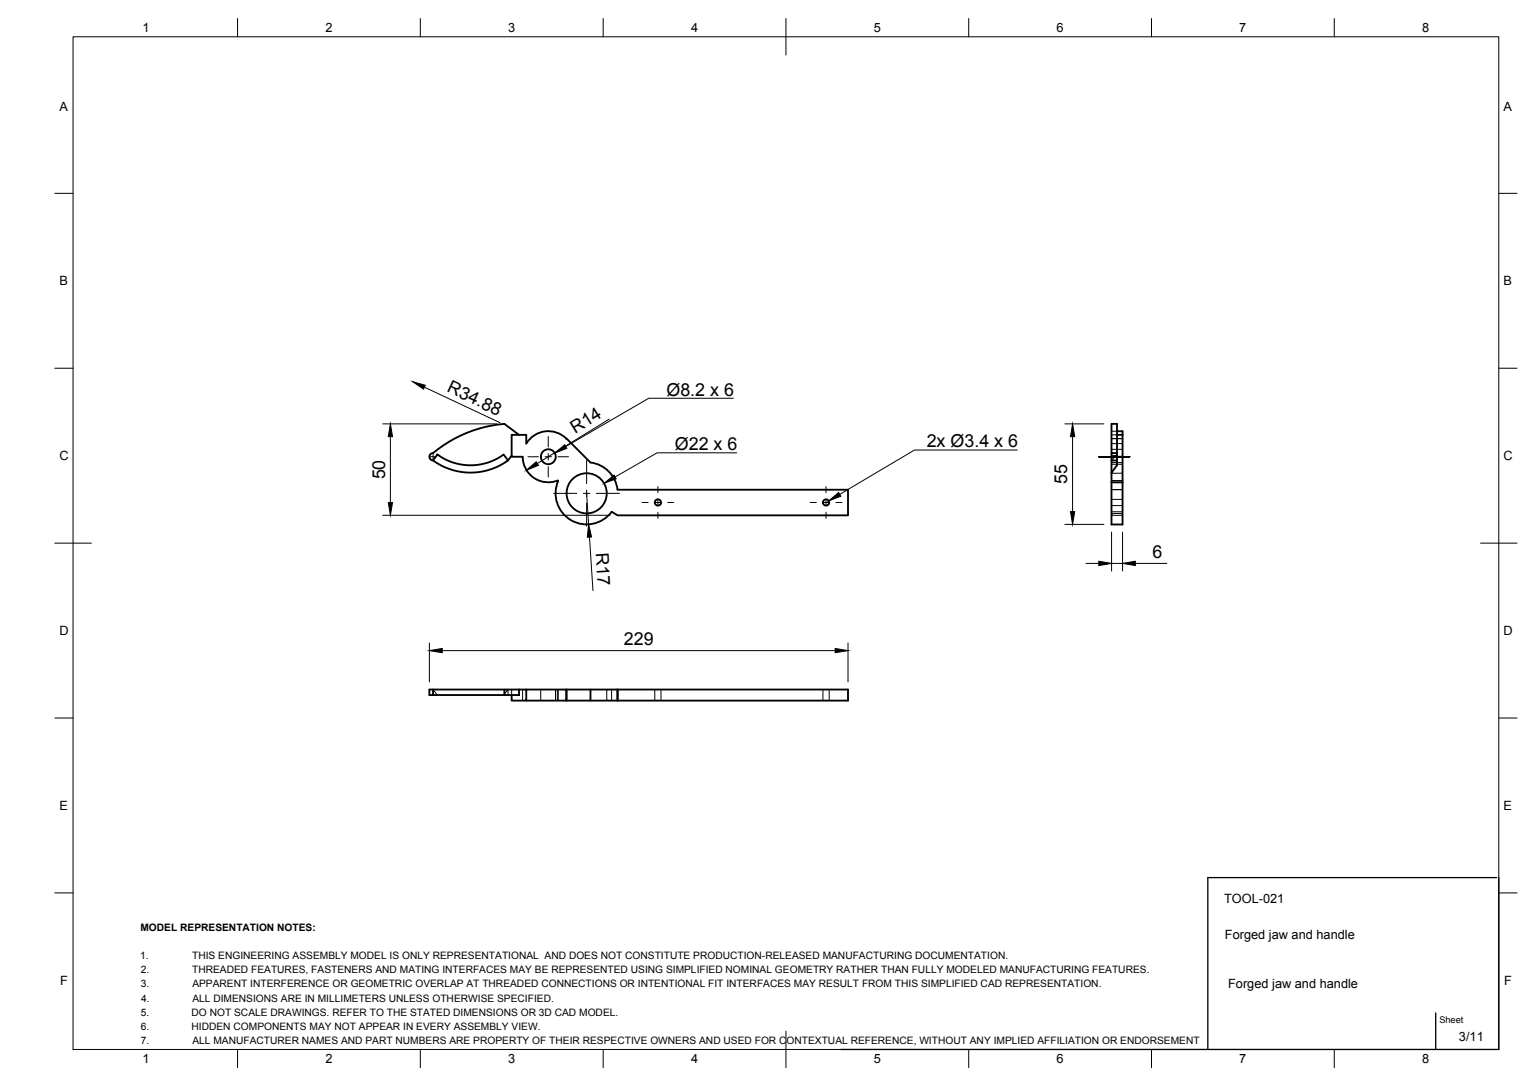
ISO-10303-21;
HEADER;
/* Generated by software containing ST-Developer
 * from STEP Tools, Inc. (www.steptools.com) 
 */

FILE_DESCRIPTION(
/* description */ (''),
/* implementation_level */ '2;1');

FILE_NAME(
/* name */ 'Forged jaw and handle.step',
/* time_stamp */ '2026-11-10T09:05:57-08:00',
/* author */ (''),
/* organization */ (''),
/* preprocessor_version */ 'ST-DEVELOPER v20.2',
/* originating_system */ 'Autodesk Translation Framework v15.17.0.0',
/* authorisation */ '');

FILE_SCHEMA (('AUTOMOTIVE_DESIGN { 1 0 10303 214 3 1 1 }'));
ENDSEC;

DATA;
#10=MECHANICAL_DESIGN_GEOMETRIC_PRESENTATION_REPRESENTATION('',(#565),#19618);
#545=SHAPE_REPRESENTATION_RELATIONSHIP('SRR','None',#19664,#555);
#555=ADVANCED_BREP_SHAPE_REPRESENTATION('',(#575),#19607);
#565=STYLED_ITEM('',(#19728),#575);
#575=MANIFOLD_SOLID_BREP('Body1',#7103);
#585=TOROIDAL_SURFACE('',#7263,1.2,0.1);
#586=TOROIDAL_SURFACE('',#7273,1.2,0.1);
#589=FACE_BOUND('',#1242,.T.);
#590=FACE_BOUND('',#1243,.T.);
#591=FACE_BOUND('',#1244,.T.);
#592=FACE_BOUND('',#1245,.T.);
#593=FACE_BOUND('',#1249,.T.);
#594=FACE_BOUND('',#1250,.T.);
#595=FACE_BOUND('',#1251,.T.);
#596=FACE_BOUND('',#1252,.T.);
#660=CONICAL_SURFACE('',#7236,3.28832599394285,0.927295218001612);
#662=PLANE('',#7235);
#663=PLANE('',#7239);
#664=PLANE('',#7240);
#665=PLANE('',#7241);
#666=PLANE('',#7248);
#667=PLANE('',#7249);
#668=PLANE('',#7250);
#669=PLANE('',#7251);
#670=PLANE('',#7252);
#671=PLANE('',#7259);
#672=PLANE('',#7270);
#673=PLANE('',#7277);
#674=PLANE('',#7278);
#675=PLANE('',#7279);
#676=PLANE('',#7280);
#677=PLANE('',#7281);
#678=PLANE('',#7282);
#679=PLANE('',#7283);
#680=PLANE('',#7284);
#821=FACE_OUTER_BOUND('',#1224,.T.);
#822=FACE_OUTER_BOUND('',#1225,.T.);
#823=FACE_OUTER_BOUND('',#1226,.T.);
#824=FACE_OUTER_BOUND('',#1227,.T.);
#825=FACE_OUTER_BOUND('',#1228,.T.);
#826=FACE_OUTER_BOUND('',#1229,.T.);
#827=FACE_OUTER_BOUND('',#1230,.T.);
#828=FACE_OUTER_BOUND('',#1231,.T.);
#829=FACE_OUTER_BOUND('',#1232,.T.);
#830=FACE_OUTER_BOUND('',#1233,.T.);
#831=FACE_OUTER_BOUND('',#1234,.T.);
#832=FACE_OUTER_BOUND('',#1235,.T.);
#833=FACE_OUTER_BOUND('',#1236,.T.);
#834=FACE_OUTER_BOUND('',#1237,.T.);
#835=FACE_OUTER_BOUND('',#1238,.T.);
#836=FACE_OUTER_BOUND('',#1239,.T.);
#837=FACE_OUTER_BOUND('',#1240,.T.);
#838=FACE_OUTER_BOUND('',#1241,.T.);
#839=FACE_OUTER_BOUND('',#1246,.T.);
#840=FACE_OUTER_BOUND('',#1247,.T.);
#841=FACE_OUTER_BOUND('',#1248,.T.);
#842=FACE_OUTER_BOUND('',#1253,.T.);
#843=FACE_OUTER_BOUND('',#1254,.T.);
#844=FACE_OUTER_BOUND('',#1255,.T.);
#845=FACE_OUTER_BOUND('',#1256,.T.);
#846=FACE_OUTER_BOUND('',#1257,.T.);
#847=FACE_OUTER_BOUND('',#1258,.T.);
#848=FACE_OUTER_BOUND('',#1259,.T.);
#849=FACE_OUTER_BOUND('',#1260,.T.);
#850=FACE_OUTER_BOUND('',#1261,.T.);
#851=FACE_OUTER_BOUND('',#1262,.T.);
#852=FACE_OUTER_BOUND('',#1263,.T.);
#1224=EDGE_LOOP('',(#4504,#4505,#4506,#4507));
#1225=EDGE_LOOP('',(#4508,#4509,#4510,#4511));
#1226=EDGE_LOOP('',(#4512,#4513,#4514,#4515));
#1227=EDGE_LOOP('',(#4516,#4517,#4518));
#1228=EDGE_LOOP('',(#4519,#4520,#4521,#4522));
#1229=EDGE_LOOP('',(#4523,#4524,#4525));
#1230=EDGE_LOOP('',(#4526,#4527,#4528,#4529));
#1231=EDGE_LOOP('',(#4530,#4531,#4532,#4533));
#1232=EDGE_LOOP('',(#4534,#4535,#4536,#4537));
#1233=EDGE_LOOP('',(#4538,#4539,#4540,#4541));
#1234=EDGE_LOOP('',(#4542,#4543,#4544,#4545,#4546,#4547,#4548,#4549,#4550));
#1235=EDGE_LOOP('',(#4551,#4552,#4553,#4554,#4555,#4556));
#1236=EDGE_LOOP('',(#4557,#4558,#4559,#4560,#4561,#4562));
#1237=EDGE_LOOP('',(#4563,#4564,#4565,#4566));
#1238=EDGE_LOOP('',(#4567,#4568,#4569,#4570));
#1239=EDGE_LOOP('',(#4571,#4572,#4573,#4574));
#1240=EDGE_LOOP('',(#4575,#4576,#4577,#4578));
#1241=EDGE_LOOP('',(#4579,#4580,#4581,#4582,#4583,#4584,#4585,#4586,#4587,
#4588,#4589,#4590,#4591,#4592,#4593,#4594));
#1242=EDGE_LOOP('',(#4595));
#1243=EDGE_LOOP('',(#4596));
#1244=EDGE_LOOP('',(#4597));
#1245=EDGE_LOOP('',(#4598));
#1246=EDGE_LOOP('',(#4599,#4600,#4601,#4602));
#1247=EDGE_LOOP('',(#4603,#4604,#4605,#4606,#4607));
#1248=EDGE_LOOP('',(#4608,#4609,#4610,#4611,#4612,#4613,#4614,#4615,#4616,
#4617,#4618,#4619,#4620,#4621,#4622,#4623,#4624,#4625,#4626,#4627,#4628));
#1249=EDGE_LOOP('',(#4629));
#1250=EDGE_LOOP('',(#4630));
#1251=EDGE_LOOP('',(#4631));
#1252=EDGE_LOOP('',(#4632));
#1253=EDGE_LOOP('',(#4633,#4634,#4635,#4636,#4637));
#1254=EDGE_LOOP('',(#4638,#4639,#4640,#4641));
#1255=EDGE_LOOP('',(#4642,#4643,#4644,#4645));
#1256=EDGE_LOOP('',(#4646,#4647,#4648,#4649));
#1257=EDGE_LOOP('',(#4650,#4651,#4652,#4653));
#1258=EDGE_LOOP('',(#4654,#4655,#4656,#4657));
#1259=EDGE_LOOP('',(#4658,#4659,#4660,#4661));
#1260=EDGE_LOOP('',(#4662,#4663,#4664,#4665));
#1261=EDGE_LOOP('',(#4666,#4667,#4668,#4669));
#1262=EDGE_LOOP('',(#4670,#4671,#4672,#4673));
#1263=EDGE_LOOP('',(#4674,#4675,#4676,#4677));
#1698=LINE('',#9324,#2157);
#1699=LINE('',#9330,#2158);
#1700=LINE('',#9336,#2159);
#1701=LINE('',#9341,#2160);
#1702=LINE('',#9343,#2161);
#1703=LINE('',#9344,#2162);
#1704=LINE('',#9348,#2163);
#1705=LINE('',#9353,#2164);
#1706=LINE('',#9354,#2165);
#1707=LINE('',#9358,#2166);
#1708=LINE('',#9359,#2167);
#1709=LINE('',#9360,#2168);
#1710=LINE('',#9364,#2169);
#1711=LINE('',#9366,#2170);
#1712=LINE('',#9368,#2171);
#1713=LINE('',#9369,#2172);
#1714=LINE('',#9375,#2173);
#1715=LINE('',#9381,#2174);
#1716=LINE('',#9382,#2175);
#1717=LINE('',#9385,#2176);
#1718=LINE('',#9387,#2177);
#1719=LINE('',#9389,#2178);
#1720=LINE('',#9390,#2179);
#1721=LINE('',#9393,#2180);
#1722=LINE('',#9395,#2181);
#1723=LINE('',#9396,#2182);
#1724=LINE('',#9400,#2183);
#1725=LINE('',#9401,#2184);
#1726=LINE('',#9402,#2185);
#1727=LINE('',#9406,#2186);
#1728=LINE('',#9407,#2187);
#1729=LINE('',#9408,#2188);
#1730=LINE('',#9413,#2189);
#1731=LINE('',#9419,#2190);
#1732=LINE('',#9423,#2191);
#1733=LINE('',#9427,#2192);
#1734=LINE('',#9429,#2193);
#1735=LINE('',#9431,#2194);
#1736=LINE('',#9433,#2195);
#1737=LINE('',#9435,#2196);
#1738=LINE('',#9439,#2197);
#1739=LINE('',#9440,#2198);
#1740=LINE('',#9454,#2199);
#1741=LINE('',#9457,#2200);
#1742=LINE('',#9459,#2201);
#1743=LINE('',#9463,#2202);
#1744=LINE('',#9465,#2203);
#1745=LINE('',#9467,#2204);
#1746=LINE('',#9469,#2205);
#1747=LINE('',#9471,#2206);
#1748=LINE('',#9474,#2207);
#1749=LINE('',#9478,#2208);
#1750=LINE('',#9479,#2209);
#1751=LINE('',#9481,#2210);
#1752=LINE('',#9482,#2211);
#1753=LINE('',#9484,#2212);
#1754=LINE('',#9486,#2213);
#1755=LINE('',#9489,#2214);
#1756=LINE('',#9492,#2215);
#1757=LINE('',#9494,#2216);
#2157=VECTOR('',#7777,0.17);
#2158=VECTOR('',#7784,0.17);
#2159=VECTOR('',#7791,0.41);
#2160=VECTOR('',#7796,1.);
#2161=VECTOR('',#7797,1.);
#2162=VECTOR('',#7798,1.);
#2163=VECTOR('',#7801,1.);
#2164=VECTOR('',#7808,1.);
#2165=VECTOR('',#7809,1.);
#2166=VECTOR('',#7812,1.);
#2167=VECTOR('',#7813,1.);
#2168=VECTOR('',#7814,1.);
#2169=VECTOR('',#7817,1.);
#2170=VECTOR('',#7818,1.);
#2171=VECTOR('',#7819,1.);
#2172=VECTOR('',#7820,1.);
#2173=VECTOR('',#7827,1.);
#2174=VECTOR('',#7836,1.);
#2175=VECTOR('',#7837,1.);
#2176=VECTOR('',#7840,1.);
#2177=VECTOR('',#7841,1.);
#2178=VECTOR('',#7842,1.);
#2179=VECTOR('',#7843,1.);
#2180=VECTOR('',#7846,1.);
#2181=VECTOR('',#7847,1.);
#2182=VECTOR('',#7848,1.);
#2183=VECTOR('',#7851,1.);
#2184=VECTOR('',#7852,1.);
#2185=VECTOR('',#7853,1.);
#2186=VECTOR('',#7856,1.);
#2187=VECTOR('',#7857,1.);
#2188=VECTOR('',#7858,1.);
#2189=VECTOR('',#7863,1.);
#2190=VECTOR('',#7870,1.);
#2191=VECTOR('',#7875,1.);
#2192=VECTOR('',#7878,1.);
#2193=VECTOR('',#7879,1.);
#2194=VECTOR('',#7880,1.);
#2195=VECTOR('',#7881,1.);
#2196=VECTOR('',#7882,1.);
#2197=VECTOR('',#7885,1.);
#2198=VECTOR('',#7886,1.);
#2199=VECTOR('',#7903,1.1);
#2200=VECTOR('',#7906,1.);
#2201=VECTOR('',#7907,1.);
#2202=VECTOR('',#7910,1.);
#2203=VECTOR('',#7911,1.);
#2204=VECTOR('',#7912,1.);
#2205=VECTOR('',#7913,1.);
#2206=VECTOR('',#7914,1.);
#2207=VECTOR('',#7917,1.);
#2208=VECTOR('',#7924,1.);
#2209=VECTOR('',#7925,1.);
#2210=VECTOR('',#7928,1.);
#2211=VECTOR('',#7929,1.);
#2212=VECTOR('',#7932,1.);
#2213=VECTOR('',#7935,1.);
#2214=VECTOR('',#7940,1.);
#2215=VECTOR('',#7945,1.);
#2216=VECTOR('',#7948,1.);
#2616=CIRCLE('',#7227,0.17);
#2617=CIRCLE('',#7228,0.17);
#2618=CIRCLE('',#7230,0.17);
#2619=CIRCLE('',#7231,0.17);
#2620=CIRCLE('',#7233,0.41);
#2621=CIRCLE('',#7234,0.41);
#2622=CIRCLE('',#7237,3.48832599394285);
#2623=CIRCLE('',#7238,3.08832599394285);
#2624=CIRCLE('',#7243,0.2);
#2625=CIRCLE('',#7244,0.2);
#2626=CIRCLE('',#7246,6.99668559332711);
#2627=CIRCLE('',#7247,6.99668559332711);
#2628=CIRCLE('',#7254,1.4);
#2629=CIRCLE('',#7255,1.4);
#2630=CIRCLE('',#7257,1.4);
#2631=CIRCLE('',#7258,1.4);
#2632=CIRCLE('',#7260,1.7);
#2633=CIRCLE('',#7261,1.7);
#2634=CIRCLE('',#7262,1.2);
#2635=CIRCLE('',#7264,1.2);
#2636=CIRCLE('',#7265,0.1);
#2637=CIRCLE('',#7266,1.1);
#2638=CIRCLE('',#7268,1.1);
#2639=CIRCLE('',#7269,1.1);
#2640=CIRCLE('',#7271,1.7);
#2641=CIRCLE('',#7272,1.7);
#2642=CIRCLE('',#7274,0.1);
#2810=VERTEX_POINT('',#9321);
#2811=VERTEX_POINT('',#9323);
#2812=VERTEX_POINT('',#9327);
#2813=VERTEX_POINT('',#9329);
#2814=VERTEX_POINT('',#9333);
#2815=VERTEX_POINT('',#9335);
#2816=VERTEX_POINT('',#9339);
#2817=VERTEX_POINT('',#9340);
#2818=VERTEX_POINT('',#9342);
#2819=VERTEX_POINT('',#9346);
#2820=VERTEX_POINT('',#9347);
#2821=VERTEX_POINT('',#9352);
#2822=VERTEX_POINT('',#9356);
#2823=VERTEX_POINT('',#9357);
#2824=VERTEX_POINT('',#9362);
#2825=VERTEX_POINT('',#9363);
#2826=VERTEX_POINT('',#9365);
#2827=VERTEX_POINT('',#9367);
#2828=VERTEX_POINT('',#9371);
#2829=VERTEX_POINT('',#9373);
#2830=VERTEX_POINT('',#9380);
#2831=VERTEX_POINT('',#9384);
#2832=VERTEX_POINT('',#9386);
#2833=VERTEX_POINT('',#9388);
#2834=VERTEX_POINT('',#9392);
#2835=VERTEX_POINT('',#9394);
#2836=VERTEX_POINT('',#9398);
#2837=VERTEX_POINT('',#9399);
#2838=VERTEX_POINT('',#9404);
#2839=VERTEX_POINT('',#9405);
#2840=VERTEX_POINT('',#9410);
#2841=VERTEX_POINT('',#9412);
#2842=VERTEX_POINT('',#9416);
#2843=VERTEX_POINT('',#9418);
#2844=VERTEX_POINT('',#9422);
#2845=VERTEX_POINT('',#9424);
#2846=VERTEX_POINT('',#9426);
#2847=VERTEX_POINT('',#9428);
#2848=VERTEX_POINT('',#9430);
#2849=VERTEX_POINT('',#9432);
#2850=VERTEX_POINT('',#9434);
#2851=VERTEX_POINT('',#9436);
#2852=VERTEX_POINT('',#9438);
#2853=VERTEX_POINT('',#9441);
#2854=VERTEX_POINT('',#9444);
#2855=VERTEX_POINT('',#9446);
#2856=VERTEX_POINT('',#9450);
#2857=VERTEX_POINT('',#9451);
#2858=VERTEX_POINT('',#9456);
#2859=VERTEX_POINT('',#9458);
#2860=VERTEX_POINT('',#9460);
#2861=VERTEX_POINT('',#9462);
#2862=VERTEX_POINT('',#9464);
#2863=VERTEX_POINT('',#9466);
#2864=VERTEX_POINT('',#9468);
#2865=VERTEX_POINT('',#9470);
#2866=VERTEX_POINT('',#9472);
#3477=EDGE_CURVE('',#2810,#2810,#2616,.T.);
#3478=EDGE_CURVE('',#2810,#2811,#1698,.T.);
#3479=EDGE_CURVE('',#2811,#2811,#2617,.T.);
#3480=EDGE_CURVE('',#2812,#2812,#2618,.T.);
#3481=EDGE_CURVE('',#2812,#2813,#1699,.T.);
#3482=EDGE_CURVE('',#2813,#2813,#2619,.T.);
#3483=EDGE_CURVE('',#2814,#2814,#2620,.T.);
#3484=EDGE_CURVE('',#2814,#2815,#1700,.T.);
#3485=EDGE_CURVE('',#2815,#2815,#2621,.T.);
#3486=EDGE_CURVE('',#2816,#2817,#1701,.T.);
#3487=EDGE_CURVE('',#2818,#2816,#1702,.T.);
#3488=EDGE_CURVE('',#2818,#2817,#1703,.T.);
#3489=EDGE_CURVE('',#2819,#2820,#1704,.T.);
#3490=EDGE_CURVE('',#2819,#2818,#2622,.T.);
#3491=EDGE_CURVE('',#2820,#2816,#2623,.T.);
#3492=EDGE_CURVE('',#2821,#2820,#1705,.T.);
#3493=EDGE_CURVE('',#2819,#2821,#1706,.T.);
#3494=EDGE_CURVE('',#2822,#2823,#1707,.T.);
#3495=EDGE_CURVE('',#2817,#2822,#1708,.T.);
#3496=EDGE_CURVE('',#2823,#2818,#1709,.T.);
#3497=EDGE_CURVE('',#2824,#2825,#1710,.T.);
#3498=EDGE_CURVE('',#2824,#2826,#1711,.T.);
#3499=EDGE_CURVE('',#2827,#2826,#1712,.T.);
#3500=EDGE_CURVE('',#2825,#2827,#1713,.T.);
#3501=EDGE_CURVE('',#2828,#2819,#2624,.T.);
#3502=EDGE_CURVE('',#2829,#2821,#2625,.T.);
#3503=EDGE_CURVE('',#2828,#2829,#1714,.T.);
#3504=EDGE_CURVE('',#2824,#2828,#2626,.T.);
#3505=EDGE_CURVE('',#2826,#2829,#2627,.T.);
#3506=EDGE_CURVE('',#2830,#2822,#1715,.T.);
#3507=EDGE_CURVE('',#2827,#2830,#1716,.T.);
#3508=EDGE_CURVE('',#2830,#2831,#1717,.T.);
#3509=EDGE_CURVE('',#2832,#2831,#1718,.T.);
#3510=EDGE_CURVE('',#2833,#2832,#1719,.T.);
#3511=EDGE_CURVE('',#2825,#2833,#1720,.T.);
#3512=EDGE_CURVE('',#2834,#2823,#1721,.T.);
#3513=EDGE_CURVE('',#2834,#2835,#1722,.T.);
#3514=EDGE_CURVE('',#2831,#2835,#1723,.T.);
#3515=EDGE_CURVE('',#2836,#2837,#1724,.T.);
#3516=EDGE_CURVE('',#2835,#2836,#1725,.T.);
#3517=EDGE_CURVE('',#2837,#2834,#1726,.T.);
#3518=EDGE_CURVE('',#2838,#2839,#1727,.T.);
#3519=EDGE_CURVE('',#2833,#2838,#1728,.T.);
#3520=EDGE_CURVE('',#2839,#2832,#1729,.T.);
#3521=EDGE_CURVE('',#2837,#2840,#2628,.T.);
#3522=EDGE_CURVE('',#2840,#2841,#1730,.T.);
#3523=EDGE_CURVE('',#2836,#2841,#2629,.T.);
#3524=EDGE_CURVE('',#2842,#2839,#2630,.T.);
#3525=EDGE_CURVE('',#2842,#2843,#1731,.T.);
#3526=EDGE_CURVE('',#2843,#2838,#2631,.T.);
#3527=EDGE_CURVE('',#2841,#2844,#1732,.T.);
#3528=EDGE_CURVE('',#2844,#2845,#2632,.T.);
#3529=EDGE_CURVE('',#2845,#2846,#1733,.T.);
#3530=EDGE_CURVE('',#2846,#2847,#1734,.T.);
#3531=EDGE_CURVE('',#2847,#2848,#1735,.T.);
#3532=EDGE_CURVE('',#2848,#2849,#1736,.T.);
#3533=EDGE_CURVE('',#2849,#2850,#1737,.T.);
#3534=EDGE_CURVE('',#2850,#2851,#2633,.T.);
#3535=EDGE_CURVE('',#2851,#2852,#1738,.T.);
#3536=EDGE_CURVE('',#2852,#2842,#1739,.T.);
#3537=EDGE_CURVE('',#2853,#2853,#2634,.T.);
#3538=EDGE_CURVE('',#2854,#2854,#2635,.T.);
#3539=EDGE_CURVE('',#2854,#2855,#2636,.T.);
#3540=EDGE_CURVE('',#2855,#2855,#2637,.T.);
#3541=EDGE_CURVE('',#2856,#2857,#2638,.T.);
#3542=EDGE_CURVE('',#2857,#2856,#2639,.T.);
#3543=EDGE_CURVE('',#2857,#2855,#1740,.T.);
#3544=EDGE_CURVE('',#2858,#2843,#1741,.T.);
#3545=EDGE_CURVE('',#2859,#2858,#1742,.T.);
#3546=EDGE_CURVE('',#2860,#2859,#2640,.T.);
#3547=EDGE_CURVE('',#2861,#2860,#1743,.T.);
#3548=EDGE_CURVE('',#2862,#2861,#1744,.T.);
#3549=EDGE_CURVE('',#2863,#2862,#1745,.T.);
#3550=EDGE_CURVE('',#2864,#2863,#1746,.T.);
#3551=EDGE_CURVE('',#2865,#2864,#1747,.T.);
#3552=EDGE_CURVE('',#2866,#2865,#2641,.T.);
#3553=EDGE_CURVE('',#2840,#2866,#1748,.T.);
#3554=EDGE_CURVE('',#2853,#2856,#2642,.T.);
#3555=EDGE_CURVE('',#2851,#2859,#1749,.T.);
#3556=EDGE_CURVE('',#2860,#2850,#1750,.T.);
#3557=EDGE_CURVE('',#2866,#2844,#1751,.T.);
#3558=EDGE_CURVE('',#2845,#2865,#1752,.T.);
#3559=EDGE_CURVE('',#2864,#2846,#1753,.T.);
#3560=EDGE_CURVE('',#2861,#2849,#1754,.T.);
#3561=EDGE_CURVE('',#2858,#2852,#1755,.T.);
#3562=EDGE_CURVE('',#2862,#2848,#1756,.T.);
#3563=EDGE_CURVE('',#2863,#2847,#1757,.T.);
#4504=ORIENTED_EDGE('',*,*,#3477,.F.);
#4505=ORIENTED_EDGE('',*,*,#3478,.T.);
#4506=ORIENTED_EDGE('',*,*,#3479,.F.);
#4507=ORIENTED_EDGE('',*,*,#3478,.F.);
#4508=ORIENTED_EDGE('',*,*,#3480,.F.);
#4509=ORIENTED_EDGE('',*,*,#3481,.T.);
#4510=ORIENTED_EDGE('',*,*,#3482,.F.);
#4511=ORIENTED_EDGE('',*,*,#3481,.F.);
#4512=ORIENTED_EDGE('',*,*,#3483,.F.);
#4513=ORIENTED_EDGE('',*,*,#3484,.T.);
#4514=ORIENTED_EDGE('',*,*,#3485,.F.);
#4515=ORIENTED_EDGE('',*,*,#3484,.F.);
#4516=ORIENTED_EDGE('',*,*,#3486,.F.);
#4517=ORIENTED_EDGE('',*,*,#3487,.F.);
#4518=ORIENTED_EDGE('',*,*,#3488,.T.);
#4519=ORIENTED_EDGE('',*,*,#3489,.F.);
#4520=ORIENTED_EDGE('',*,*,#3490,.T.);
#4521=ORIENTED_EDGE('',*,*,#3487,.T.);
#4522=ORIENTED_EDGE('',*,*,#3491,.F.);
#4523=ORIENTED_EDGE('',*,*,#3492,.F.);
#4524=ORIENTED_EDGE('',*,*,#3493,.F.);
#4525=ORIENTED_EDGE('',*,*,#3489,.T.);
#4526=ORIENTED_EDGE('',*,*,#3494,.F.);
#4527=ORIENTED_EDGE('',*,*,#3495,.F.);
#4528=ORIENTED_EDGE('',*,*,#3488,.F.);
#4529=ORIENTED_EDGE('',*,*,#3496,.F.);
#4530=ORIENTED_EDGE('',*,*,#3497,.F.);
#4531=ORIENTED_EDGE('',*,*,#3498,.T.);
#4532=ORIENTED_EDGE('',*,*,#3499,.F.);
#4533=ORIENTED_EDGE('',*,*,#3500,.F.);
#4534=ORIENTED_EDGE('',*,*,#3501,.T.);
#4535=ORIENTED_EDGE('',*,*,#3493,.T.);
#4536=ORIENTED_EDGE('',*,*,#3502,.F.);
#4537=ORIENTED_EDGE('',*,*,#3503,.F.);
#4538=ORIENTED_EDGE('',*,*,#3504,.T.);
#4539=ORIENTED_EDGE('',*,*,#3503,.T.);
#4540=ORIENTED_EDGE('',*,*,#3505,.F.);
#4541=ORIENTED_EDGE('',*,*,#3498,.F.);
#4542=ORIENTED_EDGE('',*,*,#3486,.T.);
#4543=ORIENTED_EDGE('',*,*,#3495,.T.);
#4544=ORIENTED_EDGE('',*,*,#3506,.F.);
#4545=ORIENTED_EDGE('',*,*,#3507,.F.);
#4546=ORIENTED_EDGE('',*,*,#3499,.T.);
#4547=ORIENTED_EDGE('',*,*,#3505,.T.);
#4548=ORIENTED_EDGE('',*,*,#3502,.T.);
#4549=ORIENTED_EDGE('',*,*,#3492,.T.);
#4550=ORIENTED_EDGE('',*,*,#3491,.T.);
#4551=ORIENTED_EDGE('',*,*,#3500,.T.);
#4552=ORIENTED_EDGE('',*,*,#3507,.T.);
#4553=ORIENTED_EDGE('',*,*,#3508,.T.);
#4554=ORIENTED_EDGE('',*,*,#3509,.F.);
#4555=ORIENTED_EDGE('',*,*,#3510,.F.);
#4556=ORIENTED_EDGE('',*,*,#3511,.F.);
#4557=ORIENTED_EDGE('',*,*,#3506,.T.);
#4558=ORIENTED_EDGE('',*,*,#3494,.T.);
#4559=ORIENTED_EDGE('',*,*,#3512,.F.);
#4560=ORIENTED_EDGE('',*,*,#3513,.T.);
#4561=ORIENTED_EDGE('',*,*,#3514,.F.);
#4562=ORIENTED_EDGE('',*,*,#3508,.F.);
#4563=ORIENTED_EDGE('',*,*,#3515,.F.);
#4564=ORIENTED_EDGE('',*,*,#3516,.F.);
#4565=ORIENTED_EDGE('',*,*,#3513,.F.);
#4566=ORIENTED_EDGE('',*,*,#3517,.F.);
#4567=ORIENTED_EDGE('',*,*,#3518,.F.);
#4568=ORIENTED_EDGE('',*,*,#3519,.F.);
#4569=ORIENTED_EDGE('',*,*,#3510,.T.);
#4570=ORIENTED_EDGE('',*,*,#3520,.F.);
#4571=ORIENTED_EDGE('',*,*,#3515,.T.);
#4572=ORIENTED_EDGE('',*,*,#3521,.T.);
#4573=ORIENTED_EDGE('',*,*,#3522,.T.);
#4574=ORIENTED_EDGE('',*,*,#3523,.F.);
#4575=ORIENTED_EDGE('',*,*,#3518,.T.);
#4576=ORIENTED_EDGE('',*,*,#3524,.F.);
#4577=ORIENTED_EDGE('',*,*,#3525,.T.);
#4578=ORIENTED_EDGE('',*,*,#3526,.T.);
#4579=ORIENTED_EDGE('',*,*,#3523,.T.);
#4580=ORIENTED_EDGE('',*,*,#3527,.T.);
#4581=ORIENTED_EDGE('',*,*,#3528,.T.);
#4582=ORIENTED_EDGE('',*,*,#3529,.T.);
#4583=ORIENTED_EDGE('',*,*,#3530,.T.);
#4584=ORIENTED_EDGE('',*,*,#3531,.T.);
#4585=ORIENTED_EDGE('',*,*,#3532,.T.);
#4586=ORIENTED_EDGE('',*,*,#3533,.T.);
#4587=ORIENTED_EDGE('',*,*,#3534,.T.);
#4588=ORIENTED_EDGE('',*,*,#3535,.T.);
#4589=ORIENTED_EDGE('',*,*,#3536,.T.);
#4590=ORIENTED_EDGE('',*,*,#3524,.T.);
#4591=ORIENTED_EDGE('',*,*,#3520,.T.);
#4592=ORIENTED_EDGE('',*,*,#3509,.T.);
#4593=ORIENTED_EDGE('',*,*,#3514,.T.);
#4594=ORIENTED_EDGE('',*,*,#3516,.T.);
#4595=ORIENTED_EDGE('',*,*,#3477,.T.);
#4596=ORIENTED_EDGE('',*,*,#3480,.T.);
#4597=ORIENTED_EDGE('',*,*,#3483,.T.);
#4598=ORIENTED_EDGE('',*,*,#3537,.F.);
#4599=ORIENTED_EDGE('',*,*,#3538,.T.);
#4600=ORIENTED_EDGE('',*,*,#3539,.T.);
#4601=ORIENTED_EDGE('',*,*,#3540,.T.);
#4602=ORIENTED_EDGE('',*,*,#3539,.F.);
#4603=ORIENTED_EDGE('',*,*,#3541,.F.);
#4604=ORIENTED_EDGE('',*,*,#3542,.F.);
#4605=ORIENTED_EDGE('',*,*,#3543,.T.);
#4606=ORIENTED_EDGE('',*,*,#3540,.F.);
#4607=ORIENTED_EDGE('',*,*,#3543,.F.);
#4608=ORIENTED_EDGE('',*,*,#3511,.T.);
#4609=ORIENTED_EDGE('',*,*,#3519,.T.);
#4610=ORIENTED_EDGE('',*,*,#3526,.F.);
#4611=ORIENTED_EDGE('',*,*,#3544,.F.);
#4612=ORIENTED_EDGE('',*,*,#3545,.F.);
#4613=ORIENTED_EDGE('',*,*,#3546,.F.);
#4614=ORIENTED_EDGE('',*,*,#3547,.F.);
#4615=ORIENTED_EDGE('',*,*,#3548,.F.);
#4616=ORIENTED_EDGE('',*,*,#3549,.F.);
#4617=ORIENTED_EDGE('',*,*,#3550,.F.);
#4618=ORIENTED_EDGE('',*,*,#3551,.F.);
#4619=ORIENTED_EDGE('',*,*,#3552,.F.);
#4620=ORIENTED_EDGE('',*,*,#3553,.F.);
#4621=ORIENTED_EDGE('',*,*,#3521,.F.);
#4622=ORIENTED_EDGE('',*,*,#3517,.T.);
#4623=ORIENTED_EDGE('',*,*,#3512,.T.);
#4624=ORIENTED_EDGE('',*,*,#3496,.T.);
#4625=ORIENTED_EDGE('',*,*,#3490,.F.);
#4626=ORIENTED_EDGE('',*,*,#3501,.F.);
#4627=ORIENTED_EDGE('',*,*,#3504,.F.);
#4628=ORIENTED_EDGE('',*,*,#3497,.T.);
#4629=ORIENTED_EDGE('',*,*,#3479,.T.);
#4630=ORIENTED_EDGE('',*,*,#3482,.T.);
#4631=ORIENTED_EDGE('',*,*,#3485,.T.);
#4632=ORIENTED_EDGE('',*,*,#3538,.F.);
#4633=ORIENTED_EDGE('',*,*,#3537,.T.);
#4634=ORIENTED_EDGE('',*,*,#3554,.T.);
#4635=ORIENTED_EDGE('',*,*,#3541,.T.);
#4636=ORIENTED_EDGE('',*,*,#3542,.T.);
#4637=ORIENTED_EDGE('',*,*,#3554,.F.);
#4638=ORIENTED_EDGE('',*,*,#3555,.F.);
#4639=ORIENTED_EDGE('',*,*,#3534,.F.);
#4640=ORIENTED_EDGE('',*,*,#3556,.F.);
#4641=ORIENTED_EDGE('',*,*,#3546,.T.);
#4642=ORIENTED_EDGE('',*,*,#3557,.F.);
#4643=ORIENTED_EDGE('',*,*,#3552,.T.);
#4644=ORIENTED_EDGE('',*,*,#3558,.F.);
#4645=ORIENTED_EDGE('',*,*,#3528,.F.);
#4646=ORIENTED_EDGE('',*,*,#3558,.T.);
#4647=ORIENTED_EDGE('',*,*,#3551,.T.);
#4648=ORIENTED_EDGE('',*,*,#3559,.T.);
#4649=ORIENTED_EDGE('',*,*,#3529,.F.);
#4650=ORIENTED_EDGE('',*,*,#3556,.T.);
#4651=ORIENTED_EDGE('',*,*,#3533,.F.);
#4652=ORIENTED_EDGE('',*,*,#3560,.F.);
#4653=ORIENTED_EDGE('',*,*,#3547,.T.);
#4654=ORIENTED_EDGE('',*,*,#3557,.T.);
#4655=ORIENTED_EDGE('',*,*,#3527,.F.);
#4656=ORIENTED_EDGE('',*,*,#3522,.F.);
#4657=ORIENTED_EDGE('',*,*,#3553,.T.);
#4658=ORIENTED_EDGE('',*,*,#3525,.F.);
#4659=ORIENTED_EDGE('',*,*,#3536,.F.);
#4660=ORIENTED_EDGE('',*,*,#3561,.F.);
#4661=ORIENTED_EDGE('',*,*,#3544,.T.);
#4662=ORIENTED_EDGE('',*,*,#3555,.T.);
#4663=ORIENTED_EDGE('',*,*,#3545,.T.);
#4664=ORIENTED_EDGE('',*,*,#3561,.T.);
#4665=ORIENTED_EDGE('',*,*,#3535,.F.);
#4666=ORIENTED_EDGE('',*,*,#3548,.T.);
#4667=ORIENTED_EDGE('',*,*,#3560,.T.);
#4668=ORIENTED_EDGE('',*,*,#3532,.F.);
#4669=ORIENTED_EDGE('',*,*,#3562,.F.);
#4670=ORIENTED_EDGE('',*,*,#3549,.T.);
#4671=ORIENTED_EDGE('',*,*,#3562,.T.);
#4672=ORIENTED_EDGE('',*,*,#3531,.F.);
#4673=ORIENTED_EDGE('',*,*,#3563,.F.);
#4674=ORIENTED_EDGE('',*,*,#3550,.T.);
#4675=ORIENTED_EDGE('',*,*,#3563,.T.);
#4676=ORIENTED_EDGE('',*,*,#3530,.F.);
#4677=ORIENTED_EDGE('',*,*,#3559,.F.);
#6558=CYLINDRICAL_SURFACE('',#7226,0.17);
#6559=CYLINDRICAL_SURFACE('',#7229,0.17);
#6560=CYLINDRICAL_SURFACE('',#7232,0.41);
#6561=CYLINDRICAL_SURFACE('',#7242,0.2);
#6562=CYLINDRICAL_SURFACE('',#7245,6.99668559332711);
#6563=CYLINDRICAL_SURFACE('',#7253,1.4);
#6564=CYLINDRICAL_SURFACE('',#7256,1.4);
#6565=CYLINDRICAL_SURFACE('',#7267,1.1);
#6566=CYLINDRICAL_SURFACE('',#7275,1.7);
#6567=CYLINDRICAL_SURFACE('',#7276,1.7);
#6700=ADVANCED_FACE('',(#821),#6558,.F.);
#6701=ADVANCED_FACE('',(#822),#6559,.F.);
#6702=ADVANCED_FACE('',(#823),#6560,.F.);
#6703=ADVANCED_FACE('',(#824),#662,.F.);
#6704=ADVANCED_FACE('',(#825),#660,.T.);
#6705=ADVANCED_FACE('',(#826),#663,.T.);
#6706=ADVANCED_FACE('',(#827),#664,.T.);
#6707=ADVANCED_FACE('',(#828),#665,.T.);
#6708=ADVANCED_FACE('',(#829),#6561,.T.);
#6709=ADVANCED_FACE('',(#830),#6562,.T.);
#6710=ADVANCED_FACE('',(#831),#666,.T.);
#6711=ADVANCED_FACE('',(#832),#667,.T.);
#6712=ADVANCED_FACE('',(#833),#668,.T.);
#6713=ADVANCED_FACE('',(#834),#669,.T.);
#6714=ADVANCED_FACE('',(#835),#670,.T.);
#6715=ADVANCED_FACE('',(#836),#6563,.T.);
#6716=ADVANCED_FACE('',(#837),#6564,.T.);
#6717=ADVANCED_FACE('',(#838,#589,#590,#591,#592),#671,.T.);
#6718=ADVANCED_FACE('',(#839),#585,.T.);
#6719=ADVANCED_FACE('',(#840),#6565,.F.);
#6720=ADVANCED_FACE('',(#841,#593,#594,#595,#596),#672,.F.);
#6721=ADVANCED_FACE('',(#842),#586,.T.);
#6722=ADVANCED_FACE('',(#843),#6566,.T.);
#6723=ADVANCED_FACE('',(#844),#6567,.T.);
#6724=ADVANCED_FACE('',(#845),#673,.T.);
#6725=ADVANCED_FACE('',(#846),#674,.T.);
#6726=ADVANCED_FACE('',(#847),#675,.T.);
#6727=ADVANCED_FACE('',(#848),#676,.T.);
#6728=ADVANCED_FACE('',(#849),#677,.T.);
#6729=ADVANCED_FACE('',(#850),#678,.T.);
#6730=ADVANCED_FACE('',(#851),#679,.T.);
#6731=ADVANCED_FACE('',(#852),#680,.T.);
#7103=CLOSED_SHELL('',(#6700,#6701,#6702,#6703,#6704,#6705,#6706,#6707,
#6708,#6709,#6710,#6711,#6712,#6713,#6714,#6715,#6716,#6717,#6718,#6719,
#6720,#6721,#6722,#6723,#6724,#6725,#6726,#6727,#6728,#6729,#6730,#6731));
#7225=AXIS2_PLACEMENT_3D('',#9319,#7771,#7772);
#7226=AXIS2_PLACEMENT_3D('',#9320,#7773,#7774);
#7227=AXIS2_PLACEMENT_3D('',#9322,#7775,#7776);
#7228=AXIS2_PLACEMENT_3D('',#9325,#7778,#7779);
#7229=AXIS2_PLACEMENT_3D('',#9326,#7780,#7781);
#7230=AXIS2_PLACEMENT_3D('',#9328,#7782,#7783);
#7231=AXIS2_PLACEMENT_3D('',#9331,#7785,#7786);
#7232=AXIS2_PLACEMENT_3D('',#9332,#7787,#7788);
#7233=AXIS2_PLACEMENT_3D('',#9334,#7789,#7790);
#7234=AXIS2_PLACEMENT_3D('',#9337,#7792,#7793);
#7235=AXIS2_PLACEMENT_3D('',#9338,#7794,#7795);
#7236=AXIS2_PLACEMENT_3D('',#9345,#7799,#7800);
#7237=AXIS2_PLACEMENT_3D('',#9349,#7802,#7803);
#7238=AXIS2_PLACEMENT_3D('',#9350,#7804,#7805);
#7239=AXIS2_PLACEMENT_3D('',#9351,#7806,#7807);
#7240=AXIS2_PLACEMENT_3D('',#9355,#7810,#7811);
#7241=AXIS2_PLACEMENT_3D('',#9361,#7815,#7816);
#7242=AXIS2_PLACEMENT_3D('',#9370,#7821,#7822);
#7243=AXIS2_PLACEMENT_3D('',#9372,#7823,#7824);
#7244=AXIS2_PLACEMENT_3D('',#9374,#7825,#7826);
#7245=AXIS2_PLACEMENT_3D('',#9376,#7828,#7829);
#7246=AXIS2_PLACEMENT_3D('',#9377,#7830,#7831);
#7247=AXIS2_PLACEMENT_3D('',#9378,#7832,#7833);
#7248=AXIS2_PLACEMENT_3D('',#9379,#7834,#7835);
#7249=AXIS2_PLACEMENT_3D('',#9383,#7838,#7839);
#7250=AXIS2_PLACEMENT_3D('',#9391,#7844,#7845);
#7251=AXIS2_PLACEMENT_3D('',#9397,#7849,#7850);
#7252=AXIS2_PLACEMENT_3D('',#9403,#7854,#7855);
#7253=AXIS2_PLACEMENT_3D('',#9409,#7859,#7860);
#7254=AXIS2_PLACEMENT_3D('',#9411,#7861,#7862);
#7255=AXIS2_PLACEMENT_3D('',#9414,#7864,#7865);
#7256=AXIS2_PLACEMENT_3D('',#9415,#7866,#7867);
#7257=AXIS2_PLACEMENT_3D('',#9417,#7868,#7869);
#7258=AXIS2_PLACEMENT_3D('',#9420,#7871,#7872);
#7259=AXIS2_PLACEMENT_3D('',#9421,#7873,#7874);
#7260=AXIS2_PLACEMENT_3D('',#9425,#7876,#7877);
#7261=AXIS2_PLACEMENT_3D('',#9437,#7883,#7884);
#7262=AXIS2_PLACEMENT_3D('',#9442,#7887,#7888);
#7263=AXIS2_PLACEMENT_3D('',#9443,#7889,#7890);
#7264=AXIS2_PLACEMENT_3D('',#9445,#7891,#7892);
#7265=AXIS2_PLACEMENT_3D('',#9447,#7893,#7894);
#7266=AXIS2_PLACEMENT_3D('',#9448,#7895,#7896);
#7267=AXIS2_PLACEMENT_3D('',#9449,#7897,#7898);
#7268=AXIS2_PLACEMENT_3D('',#9452,#7899,#7900);
#7269=AXIS2_PLACEMENT_3D('',#9453,#7901,#7902);
#7270=AXIS2_PLACEMENT_3D('',#9455,#7904,#7905);
#7271=AXIS2_PLACEMENT_3D('',#9461,#7908,#7909);
#7272=AXIS2_PLACEMENT_3D('',#9473,#7915,#7916);
#7273=AXIS2_PLACEMENT_3D('',#9475,#7918,#7919);
#7274=AXIS2_PLACEMENT_3D('',#9476,#7920,#7921);
#7275=AXIS2_PLACEMENT_3D('',#9477,#7922,#7923);
#7276=AXIS2_PLACEMENT_3D('',#9480,#7926,#7927);
#7277=AXIS2_PLACEMENT_3D('',#9483,#7930,#7931);
#7278=AXIS2_PLACEMENT_3D('',#9485,#7933,#7934);
#7279=AXIS2_PLACEMENT_3D('',#9487,#7936,#7937);
#7280=AXIS2_PLACEMENT_3D('',#9488,#7938,#7939);
#7281=AXIS2_PLACEMENT_3D('',#9490,#7941,#7942);
#7282=AXIS2_PLACEMENT_3D('',#9491,#7943,#7944);
#7283=AXIS2_PLACEMENT_3D('',#9493,#7946,#7947);
#7284=AXIS2_PLACEMENT_3D('',#9495,#7949,#7950);
#7771=DIRECTION('axis',(0.,0.,1.));
#7772=DIRECTION('refdir',(1.,0.,0.));
#7773=DIRECTION('center_axis',(0.,0.,-1.));
#7774=DIRECTION('ref_axis',(1.,0.,0.));
#7775=DIRECTION('center_axis',(0.,0.,-1.));
#7776=DIRECTION('ref_axis',(1.,0.,0.));
#7777=DIRECTION('',(0.,0.,-1.));
#7778=DIRECTION('center_axis',(0.,0.,1.));
#7779=DIRECTION('ref_axis',(1.,0.,0.));
#7780=DIRECTION('center_axis',(0.,0.,-1.));
#7781=DIRECTION('ref_axis',(1.,0.,0.));
#7782=DIRECTION('center_axis',(0.,0.,-1.));
#7783=DIRECTION('ref_axis',(1.,0.,0.));
#7784=DIRECTION('',(0.,0.,-1.));
#7785=DIRECTION('center_axis',(0.,0.,1.));
#7786=DIRECTION('ref_axis',(1.,0.,0.));
#7787=DIRECTION('center_axis',(0.,0.,-1.));
#7788=DIRECTION('ref_axis',(1.,0.,0.));
#7789=DIRECTION('center_axis',(0.,0.,-1.));
#7790=DIRECTION('ref_axis',(1.,0.,0.));
#7791=DIRECTION('',(0.,0.,-1.));
#7792=DIRECTION('center_axis',(0.,0.,1.));
#7793=DIRECTION('ref_axis',(1.,0.,0.));
#7794=DIRECTION('center_axis',(0.809097497835397,0.587674432825267,5.7205382811039E-17));
#7795=DIRECTION('ref_axis',(1.84528382722603E-17,-1.22747433027317E-16,
1.));
#7796=DIRECTION('',(0.587674432825267,-0.809097497835397,0.));
#7797=DIRECTION('',(-0.470139546260214,0.647277998268318,0.6));
#7798=DIRECTION('',(0.,0.,1.));
#7799=DIRECTION('center_axis',(0.,0.,-1.));
#7800=DIRECTION('ref_axis',(-0.587674432825267,-0.809097497835397,0.));
#7801=DIRECTION('',(0.470139546260214,0.647277998268318,0.6));
#7802=DIRECTION('center_axis',(0.,0.,1.));
#7803=DIRECTION('ref_axis',(-0.587674432825267,-0.809097497835397,0.));
#7804=DIRECTION('center_axis',(0.,0.,1.));
#7805=DIRECTION('ref_axis',(-0.587674432825267,-0.809097497835397,0.));
#7806=DIRECTION('center_axis',(0.809097497835397,-0.587674432825267,5.7205382811039E-17));
#7807=DIRECTION('ref_axis',(-1.11022302462516E-16,-5.55111512312578E-17,
1.));
#7808=DIRECTION('',(0.587674432825267,0.809097497835397,0.));
#7809=DIRECTION('',(0.,0.,1.));
#7810=DIRECTION('center_axis',(0.8,-0.6,0.));
#7811=DIRECTION('ref_axis',(0.6,0.8,0.));
#7812=DIRECTION('',(0.,0.,-1.));
#7813=DIRECTION('',(0.6,0.8,0.));
#7814=DIRECTION('',(-0.6,-0.8,0.));
#7815=DIRECTION('center_axis',(0.6,0.8,0.));
#7816=DIRECTION('ref_axis',(-0.8,0.6,0.));
#7817=DIRECTION('',(0.8,-0.6,0.));
#7818=DIRECTION('',(0.,0.,1.));
#7819=DIRECTION('',(-0.8,0.6,0.));
#7820=DIRECTION('',(0.,0.,1.));
#7821=DIRECTION('center_axis',(0.,0.,1.));
#7822=DIRECTION('ref_axis',(4.44089209850063E-15,1.,0.));
#7823=DIRECTION('center_axis',(0.,0.,1.));
#7824=DIRECTION('ref_axis',(4.44089209850063E-15,1.,0.));
#7825=DIRECTION('center_axis',(0.,0.,1.));
#7826=DIRECTION('ref_axis',(4.44089209850063E-15,1.,0.));
#7827=DIRECTION('',(0.,0.,1.));
#7828=DIRECTION('center_axis',(0.,0.,1.));
#7829=DIRECTION('ref_axis',(-0.0832212223210449,0.996531097435194,0.));
#7830=DIRECTION('center_axis',(0.,0.,1.));
#7831=DIRECTION('ref_axis',(-0.0832212223210449,0.996531097435194,0.));
#7832=DIRECTION('center_axis',(0.,0.,1.));
#7833=DIRECTION('ref_axis',(-0.0832212223210449,0.996531097435194,0.));
#7834=DIRECTION('center_axis',(0.,0.,1.));
#7835=DIRECTION('ref_axis',(1.,0.,0.));
#7836=DIRECTION('',(0.,-1.,0.));
#7837=DIRECTION('',(-1.,0.,0.));
#7838=DIRECTION('center_axis',(0.,1.,0.));
#7839=DIRECTION('ref_axis',(-1.,0.,0.));
#7840=DIRECTION('',(0.,0.,1.));
#7841=DIRECTION('',(-1.,0.,0.));
#7842=DIRECTION('',(0.,0.,1.));
#7843=DIRECTION('',(1.,0.,0.));
#7844=DIRECTION('center_axis',(-1.,0.,0.));
#7845=DIRECTION('ref_axis',(0.,-1.,0.));
#7846=DIRECTION('',(0.,1.,0.));
#7847=DIRECTION('',(0.,0.,1.));
#7848=DIRECTION('',(0.,-1.,0.));
#7849=DIRECTION('center_axis',(0.,-1.,0.));
#7850=DIRECTION('ref_axis',(1.,0.,0.));
#7851=DIRECTION('',(0.,0.,-1.));
#7852=DIRECTION('',(1.,0.,0.));
#7853=DIRECTION('',(-1.,0.,0.));
#7854=DIRECTION('center_axis',(1.,0.,0.));
#7855=DIRECTION('ref_axis',(0.,1.,0.));
#7856=DIRECTION('',(0.,0.,1.));
#7857=DIRECTION('',(0.,-1.,0.));
#7858=DIRECTION('',(0.,1.,0.));
#7859=DIRECTION('center_axis',(0.,0.,1.));
#7860=DIRECTION('ref_axis',(1.,0.,0.));
#7861=DIRECTION('center_axis',(0.,0.,1.));
#7862=DIRECTION('ref_axis',(1.,0.,0.));
#7863=DIRECTION('',(0.,0.,1.));
#7864=DIRECTION('center_axis',(0.,0.,1.));
#7865=DIRECTION('ref_axis',(1.,0.,0.));
#7866=DIRECTION('center_axis',(0.,0.,1.));
#7867=DIRECTION('ref_axis',(1.,0.,0.));
#7868=DIRECTION('center_axis',(0.,0.,1.));
#7869=DIRECTION('ref_axis',(1.,0.,0.));
#7870=DIRECTION('',(0.,0.,-1.));
#7871=DIRECTION('center_axis',(0.,0.,1.));
#7872=DIRECTION('ref_axis',(1.,0.,0.));
#7873=DIRECTION('center_axis',(0.,0.,1.));
#7874=DIRECTION('ref_axis',(1.,0.,0.));
#7875=DIRECTION('',(0.865426285481126,-0.501036270541705,0.));
#7876=DIRECTION('center_axis',(0.,0.,1.));
#7877=DIRECTION('ref_axis',(1.,0.,0.));
#7878=DIRECTION('',(0.865426285481126,-0.501036270541705,0.));
#7879=DIRECTION('',(1.,0.,0.));
#7880=DIRECTION('',(0.,1.,0.));
#7881=DIRECTION('',(-1.,0.,0.));
#7882=DIRECTION('',(-0.707106781186548,0.707106781186548,0.));
#7883=DIRECTION('center_axis',(0.,0.,1.));
#7884=DIRECTION('ref_axis',(1.,0.,0.));
#7885=DIRECTION('',(-0.707106781186548,0.707106781186548,0.));
#7886=DIRECTION('',(-0.447213595499958,-0.894427190999916,0.));
#7887=DIRECTION('center_axis',(0.,0.,1.));
#7888=DIRECTION('ref_axis',(-1.,0.,0.));
#7889=DIRECTION('center_axis',(0.,0.,1.));
#7890=DIRECTION('ref_axis',(1.,0.,0.));
#7891=DIRECTION('center_axis',(0.,0.,-1.));
#7892=DIRECTION('ref_axis',(-1.,2.01858731750028E-16,0.));
#7893=DIRECTION('center_axis',(0.,-1.,0.));
#7894=DIRECTION('ref_axis',(-1.,0.,0.));
#7895=DIRECTION('center_axis',(0.,0.,1.));
#7896=DIRECTION('ref_axis',(-1.,2.01858731750028E-16,0.));
#7897=DIRECTION('center_axis',(0.,0.,-1.));
#7898=DIRECTION('ref_axis',(1.,0.,0.));
#7899=DIRECTION('center_axis',(0.,0.,-1.));
#7900=DIRECTION('ref_axis',(-1.,0.,0.));
#7901=DIRECTION('center_axis',(0.,0.,-1.));
#7902=DIRECTION('ref_axis',(-1.,0.,0.));
#7903=DIRECTION('',(0.,0.,-1.));
#7904=DIRECTION('center_axis',(0.,0.,1.));
#7905=DIRECTION('ref_axis',(1.,0.,0.));
#7906=DIRECTION('',(-0.447213595499958,-0.894427190999916,0.));
#7907=DIRECTION('',(-0.707106781186548,0.707106781186548,0.));
#7908=DIRECTION('center_axis',(0.,0.,1.));
#7909=DIRECTION('ref_axis',(1.,0.,0.));
#7910=DIRECTION('',(-0.707106781186548,0.707106781186548,0.));
#7911=DIRECTION('',(-1.,0.,0.));
#7912=DIRECTION('',(0.,1.,0.));
#7913=DIRECTION('',(1.,0.,0.));
#7914=DIRECTION('',(0.865426285481126,-0.501036270541705,0.));
#7915=DIRECTION('center_axis',(0.,0.,1.));
#7916=DIRECTION('ref_axis',(1.,0.,0.));
#7917=DIRECTION('',(0.865426285481126,-0.501036270541705,0.));
#7918=DIRECTION('center_axis',(0.,0.,-1.));
#7919=DIRECTION('ref_axis',(-1.,0.,0.));
#7920=DIRECTION('center_axis',(0.,-1.,0.));
#7921=DIRECTION('ref_axis',(1.,0.,0.));
#7922=DIRECTION('center_axis',(0.,0.,1.));
#7923=DIRECTION('ref_axis',(1.,0.,0.));
#7924=DIRECTION('',(0.,0.,-1.));
#7925=DIRECTION('',(0.,0.,1.));
#7926=DIRECTION('center_axis',(0.,0.,1.));
#7927=DIRECTION('ref_axis',(-0.501036270541705,-0.865426285481126,0.));
#7928=DIRECTION('',(0.,0.,1.));
#7929=DIRECTION('',(0.,0.,-1.));
#7930=DIRECTION('center_axis',(-0.501036270541705,-0.865426285481126,0.));
#7931=DIRECTION('ref_axis',(0.865426285481126,-0.501036270541705,0.));
#7932=DIRECTION('',(0.,0.,1.));
#7933=DIRECTION('center_axis',(0.707106781186548,0.707106781186548,0.));
#7934=DIRECTION('ref_axis',(-0.707106781186548,0.707106781186548,0.));
#7935=DIRECTION('',(0.,0.,1.));
#7936=DIRECTION('center_axis',(-0.501036270541705,-0.865426285481126,0.));
#7937=DIRECTION('ref_axis',(0.865426285481126,-0.501036270541705,0.));
#7938=DIRECTION('center_axis',(-0.894427190999916,0.447213595499958,0.));
#7939=DIRECTION('ref_axis',(-0.447213595499958,-0.894427190999916,0.));
#7940=DIRECTION('',(0.,0.,1.));
#7941=DIRECTION('center_axis',(0.707106781186548,0.707106781186548,0.));
#7942=DIRECTION('ref_axis',(-0.707106781186548,0.707106781186548,0.));
#7943=DIRECTION('center_axis',(0.,1.,0.));
#7944=DIRECTION('ref_axis',(-1.,0.,0.));
#7945=DIRECTION('',(0.,0.,1.));
#7946=DIRECTION('center_axis',(1.,0.,0.));
#7947=DIRECTION('ref_axis',(0.,1.,0.));
#7948=DIRECTION('',(0.,0.,1.));
#7949=DIRECTION('center_axis',(0.,-1.,0.));
#7950=DIRECTION('ref_axis',(1.,0.,0.));
#9319=CARTESIAN_POINT('',(0.,0.,0.));
#9320=CARTESIAN_POINT('Origin',(6.,-2.5,0.3));
#9321=CARTESIAN_POINT('',(5.83,-2.5,0.6));
#9322=CARTESIAN_POINT('Origin',(6.,-2.5,0.6));
#9323=CARTESIAN_POINT('',(5.83,-2.5,0.));
#9324=CARTESIAN_POINT('',(5.83,-2.5,0.3));
#9325=CARTESIAN_POINT('Origin',(6.,-2.5,0.));
#9326=CARTESIAN_POINT('Origin',(15.2,-2.5,0.3));
#9327=CARTESIAN_POINT('',(15.03,-2.5,0.6));
#9328=CARTESIAN_POINT('Origin',(15.2,-2.5,0.6));
#9329=CARTESIAN_POINT('',(15.03,-2.5,0.));
#9330=CARTESIAN_POINT('',(15.03,-2.5,0.3));
#9331=CARTESIAN_POINT('Origin',(15.2,-2.5,0.));
#9332=CARTESIAN_POINT('Origin',(0.,0.,0.3));
#9333=CARTESIAN_POINT('',(-0.41,5.02105187650415E-17,0.6));
#9334=CARTESIAN_POINT('Origin',(0.,0.,0.6));
#9335=CARTESIAN_POINT('',(-0.41,5.02105187650415E-17,0.));
#9336=CARTESIAN_POINT('',(-0.41,5.02105187650415E-17,0.3));
#9337=CARTESIAN_POINT('Origin',(0.,0.,0.));
#9338=CARTESIAN_POINT('Origin',(-2.30284302574442,-0.0584079378788056,0.175));
#9339=CARTESIAN_POINT('',(-2.43506977313011,0.123638999134158,0.3));
#9340=CARTESIAN_POINT('',(-2.2,-0.2,0.3));
#9341=CARTESIAN_POINT('',(-2.72946351288801,0.528953957403482,0.3));
#9342=CARTESIAN_POINT('',(-2.2,-0.2,0.));
#9343=CARTESIAN_POINT('',(-2.2,-0.2,-4.89203798331893E-32));
#9344=CARTESIAN_POINT('',(-2.2,-0.2,0.));
#9345=CARTESIAN_POINT('Origin',(-4.25,2.62239583333333,0.15));
#9346=CARTESIAN_POINT('',(-6.3,-0.2,0.));
#9347=CARTESIAN_POINT('',(-6.06493022686989,0.123638999134159,0.3));
#9348=CARTESIAN_POINT('',(-6.3,-0.2,-4.89203798331893E-32));
#9349=CARTESIAN_POINT('Origin',(-4.25,2.62239583333333,0.));
#9350=CARTESIAN_POINT('Origin',(-4.25,2.62239583333333,0.3));
#9351=CARTESIAN_POINT('Origin',(-6.19715697425558,-0.0584079378788055,0.175));
#9352=CARTESIAN_POINT('',(-6.3,-0.2,0.3));
#9353=CARTESIAN_POINT('',(-5.70146423931269,0.624051140031634,0.3));
#9354=CARTESIAN_POINT('',(-6.3,-0.2,0.));
#9355=CARTESIAN_POINT('Origin',(-2.2,-0.2,0.));
#9356=CARTESIAN_POINT('',(-2.,0.0666666666666669,0.3));
#9357=CARTESIAN_POINT('',(-2.,0.0666666666666669,0.));
#9358=CARTESIAN_POINT('',(-2.,0.0666666666666667,0.));
#9359=CARTESIAN_POINT('',(-1.6,0.6,0.3));
#9360=CARTESIAN_POINT('',(-1.6,0.6,0.));
#9361=CARTESIAN_POINT('Origin',(-1.6,1.2,0.));
#9362=CARTESIAN_POINT('',(-2.4,1.8,0.));
#9363=CARTESIAN_POINT('',(-1.6,1.2,0.));
#9364=CARTESIAN_POINT('',(-2.4,1.8,0.));
#9365=CARTESIAN_POINT('',(-2.4,1.8,0.3));
#9366=CARTESIAN_POINT('',(-2.4,1.8,0.));
#9367=CARTESIAN_POINT('',(-1.6,1.2,0.3));
#9368=CARTESIAN_POINT('',(-2.4,1.8,0.3));
#9369=CARTESIAN_POINT('',(-1.6,1.2,0.));
#9370=CARTESIAN_POINT('Origin',(-6.3,1.38777878078145E-17,0.));
#9371=CARTESIAN_POINT('',(-6.3,0.2,0.));
#9372=CARTESIAN_POINT('Origin',(-6.3,1.38777878078145E-17,0.));
#9373=CARTESIAN_POINT('',(-6.3,0.2,0.3));
#9374=CARTESIAN_POINT('Origin',(-6.3,1.38777878078145E-17,0.3));
#9375=CARTESIAN_POINT('',(-6.3,0.2,0.));
#9376=CARTESIAN_POINT('Origin',(-1.81772727272727,-5.17241477272727,0.));
#9377=CARTESIAN_POINT('Origin',(-1.81772727272727,-5.17241477272727,0.));
#9378=CARTESIAN_POINT('Origin',(-1.81772727272727,-5.17241477272727,0.3));
#9379=CARTESIAN_POINT('Origin',(-4.05,0.467034919695243,0.3));
#9380=CARTESIAN_POINT('',(-2.,1.2,0.3));
#9381=CARTESIAN_POINT('',(-2.,0.833517459847621,0.3));
#9382=CARTESIAN_POINT('',(-2.625,1.2,0.3));
#9383=CARTESIAN_POINT('Origin',(-1.2,1.2,0.));
#9384=CARTESIAN_POINT('',(-2.,1.2,0.6));
#9385=CARTESIAN_POINT('',(-2.,1.2,0.));
#9386=CARTESIAN_POINT('',(-1.2,1.2,0.6));
#9387=CARTESIAN_POINT('',(-2.,1.2,0.6));
#9388=CARTESIAN_POINT('',(-1.2,1.2,0.));
#9389=CARTESIAN_POINT('',(-1.2,1.2,0.));
#9390=CARTESIAN_POINT('',(-2.,1.2,0.));
#9391=CARTESIAN_POINT('Origin',(-2.,1.2,0.));
#9392=CARTESIAN_POINT('',(-2.,0.,0.));
#9393=CARTESIAN_POINT('',(-2.,0.,0.));
#9394=CARTESIAN_POINT('',(-2.,0.,0.6));
#9395=CARTESIAN_POINT('',(-2.,0.,0.));
#9396=CARTESIAN_POINT('',(-2.,0.,0.6));
#9397=CARTESIAN_POINT('Origin',(-2.,0.,0.));
#9398=CARTESIAN_POINT('',(-1.4,0.,0.6));
#9399=CARTESIAN_POINT('',(-1.4,0.,0.));
#9400=CARTESIAN_POINT('',(-1.4,0.,0.));
#9401=CARTESIAN_POINT('',(-1.2,0.,0.6));
#9402=CARTESIAN_POINT('',(-1.2,0.,0.));
#9403=CARTESIAN_POINT('Origin',(-1.2,0.,0.));
#9404=CARTESIAN_POINT('',(-1.2,0.721110255092798,0.));
#9405=CARTESIAN_POINT('',(-1.2,0.721110255092798,0.6));
#9406=CARTESIAN_POINT('',(-1.2,0.721110255092798,0.));
#9407=CARTESIAN_POINT('',(-1.2,1.2,0.));
#9408=CARTESIAN_POINT('',(-1.2,1.2,0.6));
#9409=CARTESIAN_POINT('Origin',(0.,0.,0.));
#9410=CARTESIAN_POINT('',(0.518766934059614,-1.30033875129767,0.));
#9411=CARTESIAN_POINT('Origin',(0.,0.,0.));
#9412=CARTESIAN_POINT('',(0.518766934059614,-1.30033875129767,0.6));
#9413=CARTESIAN_POINT('',(0.518766934059614,-1.30033875129767,0.));
#9414=CARTESIAN_POINT('Origin',(0.,0.,0.6));
#9415=CARTESIAN_POINT('Origin',(0.,0.,0.));
#9416=CARTESIAN_POINT('',(0.993295878967653,0.986591757935306,0.6));
#9417=CARTESIAN_POINT('Origin',(0.,0.,0.6));
#9418=CARTESIAN_POINT('',(0.993295878967653,0.986591757935306,0.));
#9419=CARTESIAN_POINT('',(0.993295878967653,0.986591757935306,0.));
#9420=CARTESIAN_POINT('Origin',(0.,0.,0.));
#9421=CARTESIAN_POINT('Origin',(0.,0.,0.6));
#9422=CARTESIAN_POINT('',(0.544110909138566,-1.31501157897496,0.6));
#9423=CARTESIAN_POINT('',(0.,-1.,0.6));
#9424=CARTESIAN_POINT('',(3.46875216140085,-3.00822493554786,0.6));
#9425=CARTESIAN_POINT('Origin',(2.1,-2.,0.6));
#9426=CARTESIAN_POINT('',(3.8,-3.2,0.6));
#9427=CARTESIAN_POINT('',(0.,-1.,0.6));
#9428=CARTESIAN_POINT('',(16.4,-3.2,0.6));
#9429=CARTESIAN_POINT('',(3.8,-3.2,0.6));
#9430=CARTESIAN_POINT('',(16.4,-1.8,0.6));
#9431=CARTESIAN_POINT('',(16.4,-3.2,0.6));
#9432=CARTESIAN_POINT('',(3.8,-1.8,0.6));
#9433=CARTESIAN_POINT('',(16.4,-1.8,0.6));
#9434=CARTESIAN_POINT('',(3.78654599313281,-1.78654599313281,0.6));
#9435=CARTESIAN_POINT('',(3.8,-1.8,0.6));
#9436=CARTESIAN_POINT('',(2.31345400686719,-0.313454006867188,0.6));
#9437=CARTESIAN_POINT('Origin',(2.1,-2.,0.6));
#9438=CARTESIAN_POINT('',(1.,1.,0.6));
#9439=CARTESIAN_POINT('',(3.8,-1.8,0.6));
#9440=CARTESIAN_POINT('',(1.,1.,0.6));
#9441=CARTESIAN_POINT('',(3.3,-2.,0.6));
#9442=CARTESIAN_POINT('Origin',(2.1,-2.,0.6));
#9443=CARTESIAN_POINT('Origin',(2.1,-2.,0.1));
#9444=CARTESIAN_POINT('',(0.9,-2.,0.));
#9445=CARTESIAN_POINT('Origin',(2.1,-2.,0.));
#9446=CARTESIAN_POINT('',(1.,-2.,0.1));
#9447=CARTESIAN_POINT('Origin',(0.9,-2.,0.1));
#9448=CARTESIAN_POINT('Origin',(2.1,-2.,0.1));
#9449=CARTESIAN_POINT('Origin',(2.1,-2.,0.3));
#9450=CARTESIAN_POINT('',(3.2,-2.,0.5));
#9451=CARTESIAN_POINT('',(1.,-2.,0.5));
#9452=CARTESIAN_POINT('Origin',(2.1,-2.,0.5));
#9453=CARTESIAN_POINT('Origin',(2.1,-2.,0.5));
#9454=CARTESIAN_POINT('',(1.,-2.,0.3));
#9455=CARTESIAN_POINT('Origin',(0.,0.,0.));
#9456=CARTESIAN_POINT('',(1.,1.,0.));
#9457=CARTESIAN_POINT('',(1.,1.,0.));
#9458=CARTESIAN_POINT('',(2.31345400686719,-0.313454006867188,0.));
#9459=CARTESIAN_POINT('',(3.8,-1.8,0.));
#9460=CARTESIAN_POINT('',(3.78654599313281,-1.78654599313281,0.));
#9461=CARTESIAN_POINT('Origin',(2.1,-2.,0.));
#9462=CARTESIAN_POINT('',(3.8,-1.8,0.));
#9463=CARTESIAN_POINT('',(3.8,-1.8,0.));
#9464=CARTESIAN_POINT('',(16.4,-1.8,0.));
#9465=CARTESIAN_POINT('',(16.4,-1.8,0.));
#9466=CARTESIAN_POINT('',(16.4,-3.2,0.));
#9467=CARTESIAN_POINT('',(16.4,-3.2,0.));
#9468=CARTESIAN_POINT('',(3.8,-3.2,0.));
#9469=CARTESIAN_POINT('',(3.8,-3.2,0.));
#9470=CARTESIAN_POINT('',(3.46875216140085,-3.00822493554786,0.));
#9471=CARTESIAN_POINT('',(0.,-1.,0.));
#9472=CARTESIAN_POINT('',(0.544110909138566,-1.31501157897496,0.));
#9473=CARTESIAN_POINT('Origin',(2.1,-2.,0.));
#9474=CARTESIAN_POINT('',(0.,-1.,0.));
#9475=CARTESIAN_POINT('Origin',(2.1,-2.,0.5));
#9476=CARTESIAN_POINT('Origin',(3.3,-2.,0.5));
#9477=CARTESIAN_POINT('Origin',(2.1,-2.,0.));
#9478=CARTESIAN_POINT('',(2.31345400686719,-0.313454006867188,0.));
#9479=CARTESIAN_POINT('',(3.78654599313281,-1.78654599313281,0.));
#9480=CARTESIAN_POINT('Origin',(2.1,-2.,0.));
#9481=CARTESIAN_POINT('',(0.544110909138566,-1.31501157897496,0.));
#9482=CARTESIAN_POINT('',(3.46875216140085,-3.00822493554786,0.));
#9483=CARTESIAN_POINT('Origin',(0.,-1.,0.));
#9484=CARTESIAN_POINT('',(3.8,-3.2,0.));
#9485=CARTESIAN_POINT('Origin',(3.8,-1.8,0.));
#9486=CARTESIAN_POINT('',(3.8,-1.8,0.));
#9487=CARTESIAN_POINT('Origin',(0.,-1.,0.));
#9488=CARTESIAN_POINT('Origin',(1.,1.,0.));
#9489=CARTESIAN_POINT('',(1.,1.,0.));
#9490=CARTESIAN_POINT('Origin',(3.8,-1.8,0.));
#9491=CARTESIAN_POINT('Origin',(16.4,-1.8,0.));
#9492=CARTESIAN_POINT('',(16.4,-1.8,0.));
#9493=CARTESIAN_POINT('Origin',(16.4,-3.2,0.));
#9494=CARTESIAN_POINT('',(16.4,-3.2,0.));
#9495=CARTESIAN_POINT('Origin',(3.8,-3.2,0.));
#19594=UNCERTAINTY_MEASURE_WITH_UNIT(LENGTH_MEASURE(0.001),#19619,
'DISTANCE_ACCURACY_VALUE',
'Maximum model space distance between geometric entities at asserted c
onnectivities');
#19605=UNCERTAINTY_MEASURE_WITH_UNIT(LENGTH_MEASURE(0.001),#19619,
'DISTANCE_ACCURACY_VALUE',
'Maximum model space distance between geometric entities at asserted c
onnectivities');
#19607=(
GEOMETRIC_REPRESENTATION_CONTEXT(3)
GLOBAL_UNCERTAINTY_ASSIGNED_CONTEXT((#19594))
GLOBAL_UNIT_ASSIGNED_CONTEXT((#19619,#19621,#19622))
REPRESENTATION_CONTEXT('','3D')
);
#19618=(
GEOMETRIC_REPRESENTATION_CONTEXT(3)
GLOBAL_UNCERTAINTY_ASSIGNED_CONTEXT((#19605))
GLOBAL_UNIT_ASSIGNED_CONTEXT((#19619,#19621,#19622))
REPRESENTATION_CONTEXT('','3D')
);
#19619=(
LENGTH_UNIT()
NAMED_UNIT(*)
SI_UNIT(.CENTI.,.METRE.)
);
#19621=(
NAMED_UNIT(*)
PLANE_ANGLE_UNIT()
SI_UNIT($,.RADIAN.)
);
#19622=(
NAMED_UNIT(*)
SI_UNIT($,.STERADIAN.)
SOLID_ANGLE_UNIT()
);
#19624=SHAPE_DEFINITION_REPRESENTATION(#19636,#19664);
#19636=PRODUCT_DEFINITION_SHAPE('',$,#19677);
#19664=SHAPE_REPRESENTATION('',(#7225),#19607);
#19675=PRODUCT_DEFINITION_CONTEXT('part definition',#19713,'design');
#19677=PRODUCT_DEFINITION('Forged jaw and handle',
'Forged jaw and handle',#19689,#19675);
#19689=PRODUCT_DEFINITION_FORMATION('',$,#19716);
#19713=APPLICATION_CONTEXT(
'Core Data for Automotive Mechanical Design Process');
#19714=PRODUCT_CONTEXT('part definition',#19713,'mechanical');
#19716=PRODUCT('Forged jaw and handle','Forged jaw and handle',$,(#19714));
#19728=PRESENTATION_STYLE_ASSIGNMENT((#19736));
#19736=SURFACE_STYLE_USAGE(.BOTH.,#19744);
#19744=SURFACE_SIDE_STYLE('',(#19752));
#19752=SURFACE_STYLE_FILL_AREA(#19760);
#19760=FILL_AREA_STYLE('Tool steel gray',(#19768));
#19768=FILL_AREA_STYLE_COLOUR('Tool steel gray',#19776);
#19776=COLOUR_RGB('Tool steel gray',0.607843137254902,0.643137254901961,
0.698039215686274);
ENDSEC;
END-ISO-10303-21;
